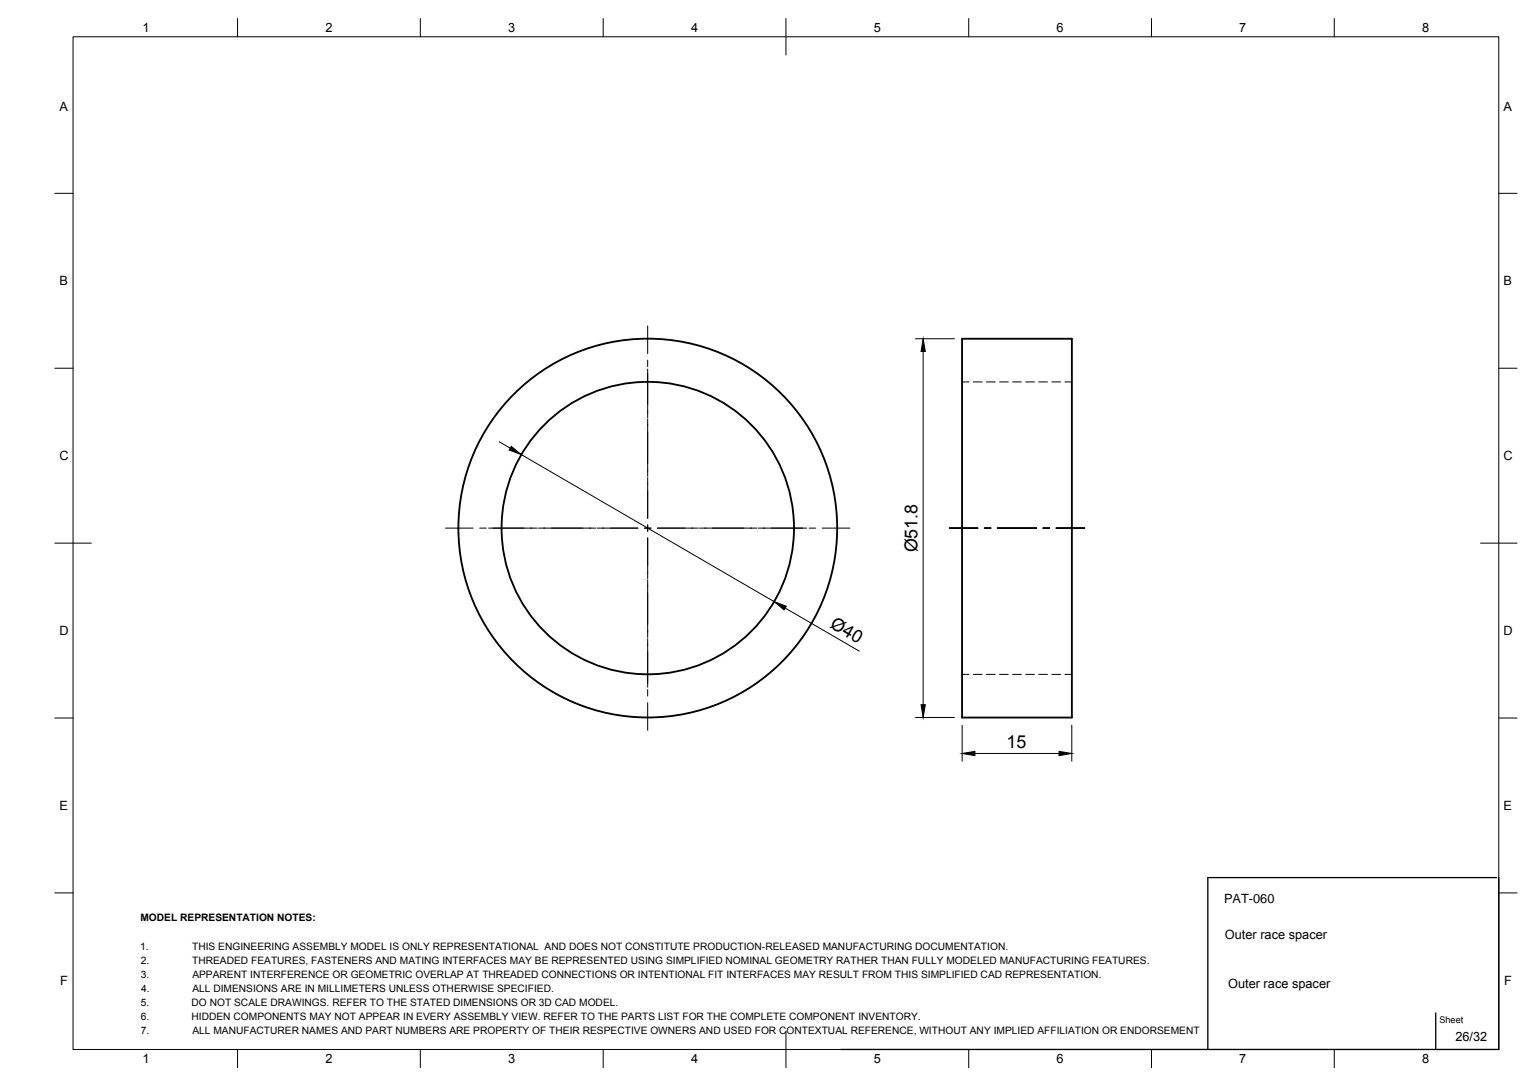
ISO-10303-21;
HEADER;
/* Generated by software containing ST-Developer
 * from STEP Tools, Inc. (www.steptools.com) 
 */

FILE_DESCRIPTION(
/* description */ ('Indexing fixture plate with plunger'),
/* implementation_level */ '2;1');

FILE_NAME(
/* name */ 'Outer race spacer.step',
/* time_stamp */ '2026-10-28T03:23:41-07:00',
/* author */ (''),
/* organization */ (''),
/* preprocessor_version */ 'ST-DEVELOPER v20.2',
/* originating_system */ 'Autodesk Translation Framework v15.17.0.0',
/* authorisation */ '');

FILE_SCHEMA (('AUTOMOTIVE_DESIGN { 1 0 10303 214 3 1 1 }'));
ENDSEC;

DATA;
#10=MECHANICAL_DESIGN_GEOMETRIC_PRESENTATION_REPRESENTATION('',(#346),#10020);
#283=SHAPE_REPRESENTATION_RELATIONSHIP('SRR','None',#10159,#310);
#310=ADVANCED_BREP_SHAPE_REPRESENTATION('',(#381),#10012);
#346=STYLED_ITEM('',(#10368),#381);
#381=MANIFOLD_SOLID_BREP('Body1',#4601);
#482=FACE_BOUND('',#1263,.T.);
#483=FACE_BOUND('',#1265,.T.);
#635=PLANE('',#5376);
#636=PLANE('',#5377);
#879=FACE_OUTER_BOUND('',#1260,.T.);
#880=FACE_OUTER_BOUND('',#1261,.T.);
#881=FACE_OUTER_BOUND('',#1262,.T.);
#882=FACE_OUTER_BOUND('',#1264,.T.);
#1260=EDGE_LOOP('',(#3841,#3842,#3843,#3844));
#1261=EDGE_LOOP('',(#3845,#3846,#3847,#3848));
#1262=EDGE_LOOP('',(#3849));
#1263=EDGE_LOOP('',(#3850));
#1264=EDGE_LOOP('',(#3851));
#1265=EDGE_LOOP('',(#3852));
#1532=LINE('',#9519,#1752);
#1533=LINE('',#9525,#1753);
#1752=VECTOR('',#6643,2.);
#1753=VECTOR('',#6650,2.59);
#2057=CIRCLE('',#5371,2.);
#2058=CIRCLE('',#5372,2.);
#2059=CIRCLE('',#5374,2.59);
#2060=CIRCLE('',#5375,2.59);
#2404=VERTEX_POINT('',#9516);
#2405=VERTEX_POINT('',#9518);
#2406=VERTEX_POINT('',#9522);
#2407=VERTEX_POINT('',#9524);
#2900=EDGE_CURVE('',#2404,#2404,#2057,.T.);
#2901=EDGE_CURVE('',#2404,#2405,#1532,.T.);
#2902=EDGE_CURVE('',#2405,#2405,#2058,.T.);
#2903=EDGE_CURVE('',#2406,#2406,#2059,.T.);
#2904=EDGE_CURVE('',#2406,#2407,#1533,.T.);
#2905=EDGE_CURVE('',#2407,#2407,#2060,.T.);
#3841=ORIENTED_EDGE('',*,*,#2900,.F.);
#3842=ORIENTED_EDGE('',*,*,#2901,.T.);
#3843=ORIENTED_EDGE('',*,*,#2902,.T.);
#3844=ORIENTED_EDGE('',*,*,#2901,.F.);
#3845=ORIENTED_EDGE('',*,*,#2903,.F.);
#3846=ORIENTED_EDGE('',*,*,#2904,.T.);
#3847=ORIENTED_EDGE('',*,*,#2905,.T.);
#3848=ORIENTED_EDGE('',*,*,#2904,.F.);
#3849=ORIENTED_EDGE('',*,*,#2903,.T.);
#3850=ORIENTED_EDGE('',*,*,#2900,.T.);
#3851=ORIENTED_EDGE('',*,*,#2905,.F.);
#3852=ORIENTED_EDGE('',*,*,#2902,.F.);
#4249=CYLINDRICAL_SURFACE('',#5370,2.);
#4250=CYLINDRICAL_SURFACE('',#5373,2.59);
#4494=ADVANCED_FACE('',(#879),#4249,.F.);
#4495=ADVANCED_FACE('',(#880),#4250,.T.);
#4496=ADVANCED_FACE('',(#881,#482),#635,.T.);
#4497=ADVANCED_FACE('',(#882,#483),#636,.F.);
#4601=CLOSED_SHELL('',(#4494,#4495,#4496,#4497));
#5369=AXIS2_PLACEMENT_3D('',#9514,#6637,#6638);
#5370=AXIS2_PLACEMENT_3D('',#9515,#6639,#6640);
#5371=AXIS2_PLACEMENT_3D('',#9517,#6641,#6642);
#5372=AXIS2_PLACEMENT_3D('',#9520,#6644,#6645);
#5373=AXIS2_PLACEMENT_3D('',#9521,#6646,#6647);
#5374=AXIS2_PLACEMENT_3D('',#9523,#6648,#6649);
#5375=AXIS2_PLACEMENT_3D('',#9526,#6651,#6652);
#5376=AXIS2_PLACEMENT_3D('',#9527,#6653,#6654);
#5377=AXIS2_PLACEMENT_3D('',#9528,#6655,#6656);
#6637=DIRECTION('axis',(0.,0.,1.));
#6638=DIRECTION('refdir',(1.,0.,0.));
#6639=DIRECTION('center_axis',(0.,0.,1.));
#6640=DIRECTION('ref_axis',(1.,0.,0.));
#6641=DIRECTION('center_axis',(0.,0.,-1.));
#6642=DIRECTION('ref_axis',(1.,0.,0.));
#6643=DIRECTION('',(0.,0.,-1.));
#6644=DIRECTION('center_axis',(0.,0.,-1.));
#6645=DIRECTION('ref_axis',(1.,0.,0.));
#6646=DIRECTION('center_axis',(0.,0.,1.));
#6647=DIRECTION('ref_axis',(1.,0.,0.));
#6648=DIRECTION('center_axis',(0.,0.,1.));
#6649=DIRECTION('ref_axis',(1.,0.,0.));
#6650=DIRECTION('',(0.,0.,-1.));
#6651=DIRECTION('center_axis',(0.,0.,1.));
#6652=DIRECTION('ref_axis',(1.,0.,0.));
#6653=DIRECTION('center_axis',(0.,0.,1.));
#6654=DIRECTION('ref_axis',(1.,0.,0.));
#6655=DIRECTION('center_axis',(0.,0.,1.));
#6656=DIRECTION('ref_axis',(1.,0.,0.));
#9514=CARTESIAN_POINT('',(0.,0.,0.));
#9515=CARTESIAN_POINT('Origin',(0.,0.,4.75));
#9516=CARTESIAN_POINT('',(-2.,-2.44929359829471E-16,6.25));
#9517=CARTESIAN_POINT('Origin',(0.,0.,6.25));
#9518=CARTESIAN_POINT('',(-2.,-2.44929359829471E-16,4.75));
#9519=CARTESIAN_POINT('',(-2.,-2.44929359829471E-16,4.75));
#9520=CARTESIAN_POINT('Origin',(0.,0.,4.75));
#9521=CARTESIAN_POINT('Origin',(0.,0.,4.75));
#9522=CARTESIAN_POINT('',(-2.59,-3.17183520979164E-16,6.25));
#9523=CARTESIAN_POINT('Origin',(0.,0.,6.25));
#9524=CARTESIAN_POINT('',(-2.59,-3.17183520979164E-16,4.75));
#9525=CARTESIAN_POINT('',(-2.59,-3.17183520979164E-16,4.75));
#9526=CARTESIAN_POINT('Origin',(0.,0.,4.75));
#9527=CARTESIAN_POINT('Origin',(0.,0.,6.25));
#9528=CARTESIAN_POINT('Origin',(0.,0.,4.75));
#9979=UNCERTAINTY_MEASURE_WITH_UNIT(LENGTH_MEASURE(0.001),#10021,
'DISTANCE_ACCURACY_VALUE',
'Maximum model space distance between geometric entities at asserted c
onnectivities');
#9987=UNCERTAINTY_MEASURE_WITH_UNIT(LENGTH_MEASURE(0.001),#10021,
'DISTANCE_ACCURACY_VALUE',
'Maximum model space distance between geometric entities at asserted c
onnectivities');
#10012=(
GEOMETRIC_REPRESENTATION_CONTEXT(3)
GLOBAL_UNCERTAINTY_ASSIGNED_CONTEXT((#9979))
GLOBAL_UNIT_ASSIGNED_CONTEXT((#10021,#10023,#10024))
REPRESENTATION_CONTEXT('','3D')
);
#10020=(
GEOMETRIC_REPRESENTATION_CONTEXT(3)
GLOBAL_UNCERTAINTY_ASSIGNED_CONTEXT((#9987))
GLOBAL_UNIT_ASSIGNED_CONTEXT((#10021,#10023,#10024))
REPRESENTATION_CONTEXT('','3D')
);
#10021=(
LENGTH_UNIT()
NAMED_UNIT(*)
SI_UNIT(.CENTI.,.METRE.)
);
#10023=(
NAMED_UNIT(*)
PLANE_ANGLE_UNIT()
SI_UNIT($,.RADIAN.)
);
#10024=(
NAMED_UNIT(*)
SI_UNIT($,.STERADIAN.)
SOLID_ANGLE_UNIT()
);
#10049=SHAPE_DEFINITION_REPRESENTATION(#10086,#10159);
#10086=PRODUCT_DEFINITION_SHAPE('',$,#10192);
#10159=SHAPE_REPRESENTATION('',(#5369),#10012);
#10167=PRODUCT_DEFINITION_CONTEXT('part definition',#10265,'design');
#10192=PRODUCT_DEFINITION('Outer race spacer','Outer race spacer',#10224,
#10167);
#10224=PRODUCT_DEFINITION_FORMATION('',$,#10291);
#10265=APPLICATION_CONTEXT(
'Core Data for Automotive Mechanical Design Process');
#10266=PRODUCT_CONTEXT('part definition',#10265,'mechanical');
#10291=PRODUCT('Outer race spacer','Outer race spacer',
'Outer race spacer',(#10266));
#10362=COLOUR_RGB('Grey',0.48,0.52,0.57);
#10363=FILL_AREA_STYLE_COLOUR('',#10362);
#10364=FILL_AREA_STYLE('',(#10363));
#10365=SURFACE_STYLE_FILL_AREA(#10364);
#10366=SURFACE_SIDE_STYLE('',(#10365));
#10367=SURFACE_STYLE_USAGE(.BOTH.,#10366);
#10368=PRESENTATION_STYLE_ASSIGNMENT((#10367));
ENDSEC;
END-ISO-10303-21;
